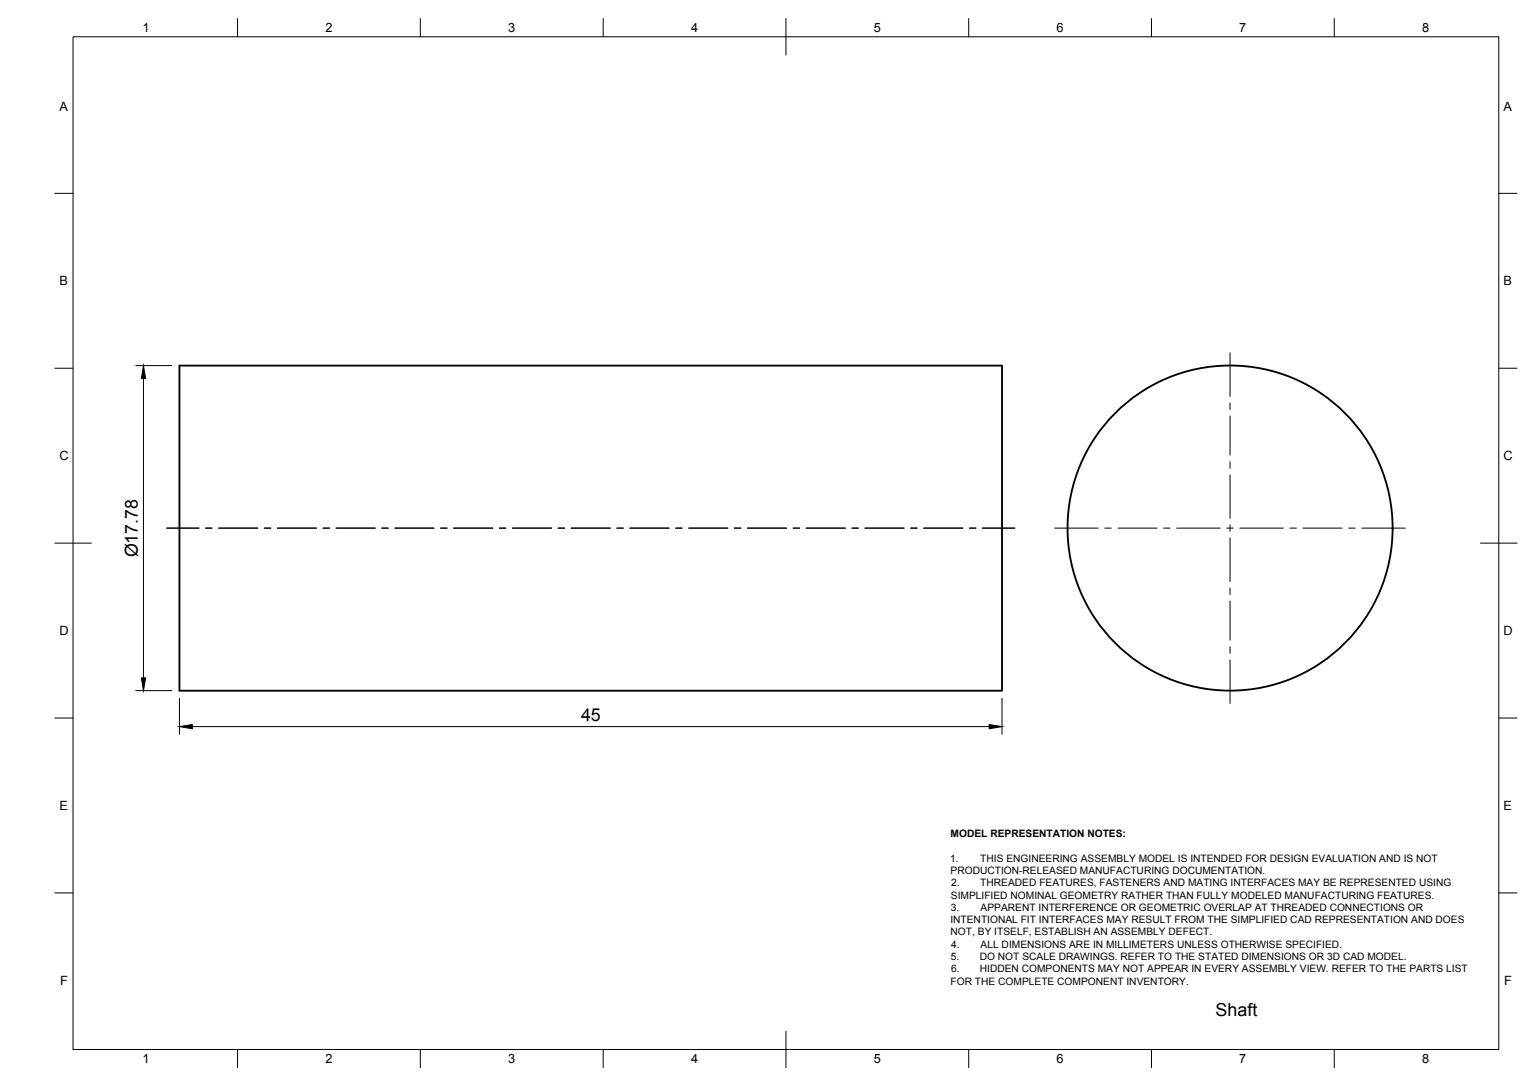
ISO-10303-21;
HEADER;
/* Generated by software containing ST-Developer
 * from STEP Tools, Inc. (www.steptools.com) 
 */

FILE_DESCRIPTION(
/* description */ ('STEP AP214'),
/* implementation_level */ '2;1');

FILE_NAME(
/* name */ 'SHAFT.step',
/* time_stamp */ '2026-10-06T11:20:11-07:00',
/* author */ (''),
/* organization */ (''),
/* preprocessor_version */ 'ST-DEVELOPER v20.2',
/* originating_system */ 'Autodesk Translation Framework v15.15.0.0',
/* authorisation */ '');

FILE_SCHEMA (('AUTOMOTIVE_DESIGN { 1 0 10303 214 3 1 1 }'));
ENDSEC;

DATA;
#10=MECHANICAL_DESIGN_GEOMETRIC_PRESENTATION_REPRESENTATION('',(#52),#2840);
#40=SHAPE_REPRESENTATION_RELATIONSHIP('SRR','None',#2871,#46);
#46=ADVANCED_BREP_SHAPE_REPRESENTATION('',(#58),#2839);
#52=STYLED_ITEM('',(#2905),#58);
#58=MANIFOLD_SOLID_BREP('Body1',#1552);
#124=PLANE('',#1833);
#125=PLANE('',#1834);
#213=FACE_OUTER_BOUND('',#331,.T.);
#214=FACE_OUTER_BOUND('',#332,.T.);
#215=FACE_OUTER_BOUND('',#333,.T.);
#331=EDGE_LOOP('',(#1400,#1401,#1402,#1403));
#332=EDGE_LOOP('',(#1404));
#333=EDGE_LOOP('',(#1405));
#426=LINE('',#2815,#519);
#519=VECTOR('',#2357,8.89);
#636=CIRCLE('',#1831,8.89);
#637=CIRCLE('',#1832,8.89);
#771=VERTEX_POINT('',#2812);
#772=VERTEX_POINT('',#2814);
#981=EDGE_CURVE('',#771,#771,#636,.T.);
#982=EDGE_CURVE('',#771,#772,#426,.T.);
#983=EDGE_CURVE('',#772,#772,#637,.T.);
#1400=ORIENTED_EDGE('',*,*,#981,.T.);
#1401=ORIENTED_EDGE('',*,*,#982,.T.);
#1402=ORIENTED_EDGE('',*,*,#983,.F.);
#1403=ORIENTED_EDGE('',*,*,#982,.F.);
#1404=ORIENTED_EDGE('',*,*,#983,.T.);
#1405=ORIENTED_EDGE('',*,*,#981,.F.);
#1456=CYLINDRICAL_SURFACE('',#1830,8.89);
#1544=ADVANCED_FACE('',(#213),#1456,.T.);
#1545=ADVANCED_FACE('',(#214),#124,.T.);
#1546=ADVANCED_FACE('',(#215),#125,.F.);
#1552=CLOSED_SHELL('',(#1544,#1545,#1546));
#1829=AXIS2_PLACEMENT_3D('',#2810,#2351,#2352);
#1830=AXIS2_PLACEMENT_3D('',#2811,#2353,#2354);
#1831=AXIS2_PLACEMENT_3D('',#2813,#2355,#2356);
#1832=AXIS2_PLACEMENT_3D('',#2816,#2358,#2359);
#1833=AXIS2_PLACEMENT_3D('',#2817,#2360,#2361);
#1834=AXIS2_PLACEMENT_3D('',#2818,#2362,#2363);
#2351=DIRECTION('axis',(0.,0.,1.));
#2352=DIRECTION('refdir',(1.,0.,0.));
#2353=DIRECTION('center_axis',(0.,-1.,0.));
#2354=DIRECTION('ref_axis',(0.,0.,-1.));
#2355=DIRECTION('center_axis',(0.,1.,0.));
#2356=DIRECTION('ref_axis',(0.,0.,1.));
#2357=DIRECTION('',(0.,1.,0.));
#2358=DIRECTION('center_axis',(0.,1.,0.));
#2359=DIRECTION('ref_axis',(0.,0.,1.));
#2360=DIRECTION('center_axis',(0.,1.,0.));
#2361=DIRECTION('ref_axis',(0.,0.,1.));
#2362=DIRECTION('center_axis',(0.,1.,0.));
#2363=DIRECTION('ref_axis',(0.,0.,1.));
#2810=CARTESIAN_POINT('',(0.,0.,0.));
#2811=CARTESIAN_POINT('Origin',(0.,45.,0.));
#2812=CARTESIAN_POINT('',(-1.088711004442E-15,0.,8.89));
#2813=CARTESIAN_POINT('Origin',(0.,0.,0.));
#2814=CARTESIAN_POINT('',(-1.088711004442E-15,45.,8.89));
#2815=CARTESIAN_POINT('',(-1.088711004442E-15,45.,8.89));
#2816=CARTESIAN_POINT('Origin',(0.,45.,0.));
#2817=CARTESIAN_POINT('Origin',(0.,45.,0.));
#2818=CARTESIAN_POINT('Origin',(0.,0.,0.));
#2831=UNCERTAINTY_MEASURE_WITH_UNIT(LENGTH_MEASURE(0.01),#2841,
'DISTANCE_ACCURACY_VALUE',
'Maximum model space distance between geometric entities at asserted c
onnectivities');
#2832=UNCERTAINTY_MEASURE_WITH_UNIT(LENGTH_MEASURE(0.01),#2841,
'DISTANCE_ACCURACY_VALUE',
'Maximum model space distance between geometric entities at asserted c
onnectivities');
#2839=(
GEOMETRIC_REPRESENTATION_CONTEXT(3)
GLOBAL_UNCERTAINTY_ASSIGNED_CONTEXT((#2831))
GLOBAL_UNIT_ASSIGNED_CONTEXT((#2841,#2843,#2844))
REPRESENTATION_CONTEXT('','3D')
);
#2840=(
GEOMETRIC_REPRESENTATION_CONTEXT(3)
GLOBAL_UNCERTAINTY_ASSIGNED_CONTEXT((#2832))
GLOBAL_UNIT_ASSIGNED_CONTEXT((#2841,#2843,#2844))
REPRESENTATION_CONTEXT('','3D')
);
#2841=(
LENGTH_UNIT()
NAMED_UNIT(*)
SI_UNIT(.MILLI.,.METRE.)
);
#2843=(
NAMED_UNIT(*)
PLANE_ANGLE_UNIT()
SI_UNIT($,.RADIAN.)
);
#2844=(
NAMED_UNIT(*)
SI_UNIT($,.STERADIAN.)
SOLID_ANGLE_UNIT()
);
#2851=SHAPE_DEFINITION_REPRESENTATION(#2858,#2871);
#2858=PRODUCT_DEFINITION_SHAPE('',$,#2879);
#2871=SHAPE_REPRESENTATION('',(#1829),#2839);
#2872=PRODUCT_DEFINITION_CONTEXT('part definition',#2895,'design');
#2879=PRODUCT_DEFINITION('Shaft','SHAFT',#2886,#2872);
#2886=PRODUCT_DEFINITION_FORMATION('',$,#2903);
#2895=APPLICATION_CONTEXT(
'Core Data for Automotive Mechanical Design Process');
#2896=PRODUCT_CONTEXT('part definition',#2895,'mechanical');
#2903=PRODUCT('Shaft','SHAFT',$,(#2896));
#2905=PRESENTATION_STYLE_ASSIGNMENT((#2907));
#2907=SURFACE_STYLE_USAGE(.BOTH.,#2909);
#2909=SURFACE_SIDE_STYLE('',(#2911));
#2911=SURFACE_STYLE_FILL_AREA(#2913);
#2913=FILL_AREA_STYLE('Opaque(202,209,238)',(#2915));
#2915=FILL_AREA_STYLE_COLOUR('Opaque(202,209,238)',#2917);
#2917=COLOUR_RGB('Opaque(202,209,238)', 0.66274510, 0.83137255, 0.94901961);
ENDSEC;
END-ISO-10303-21;
